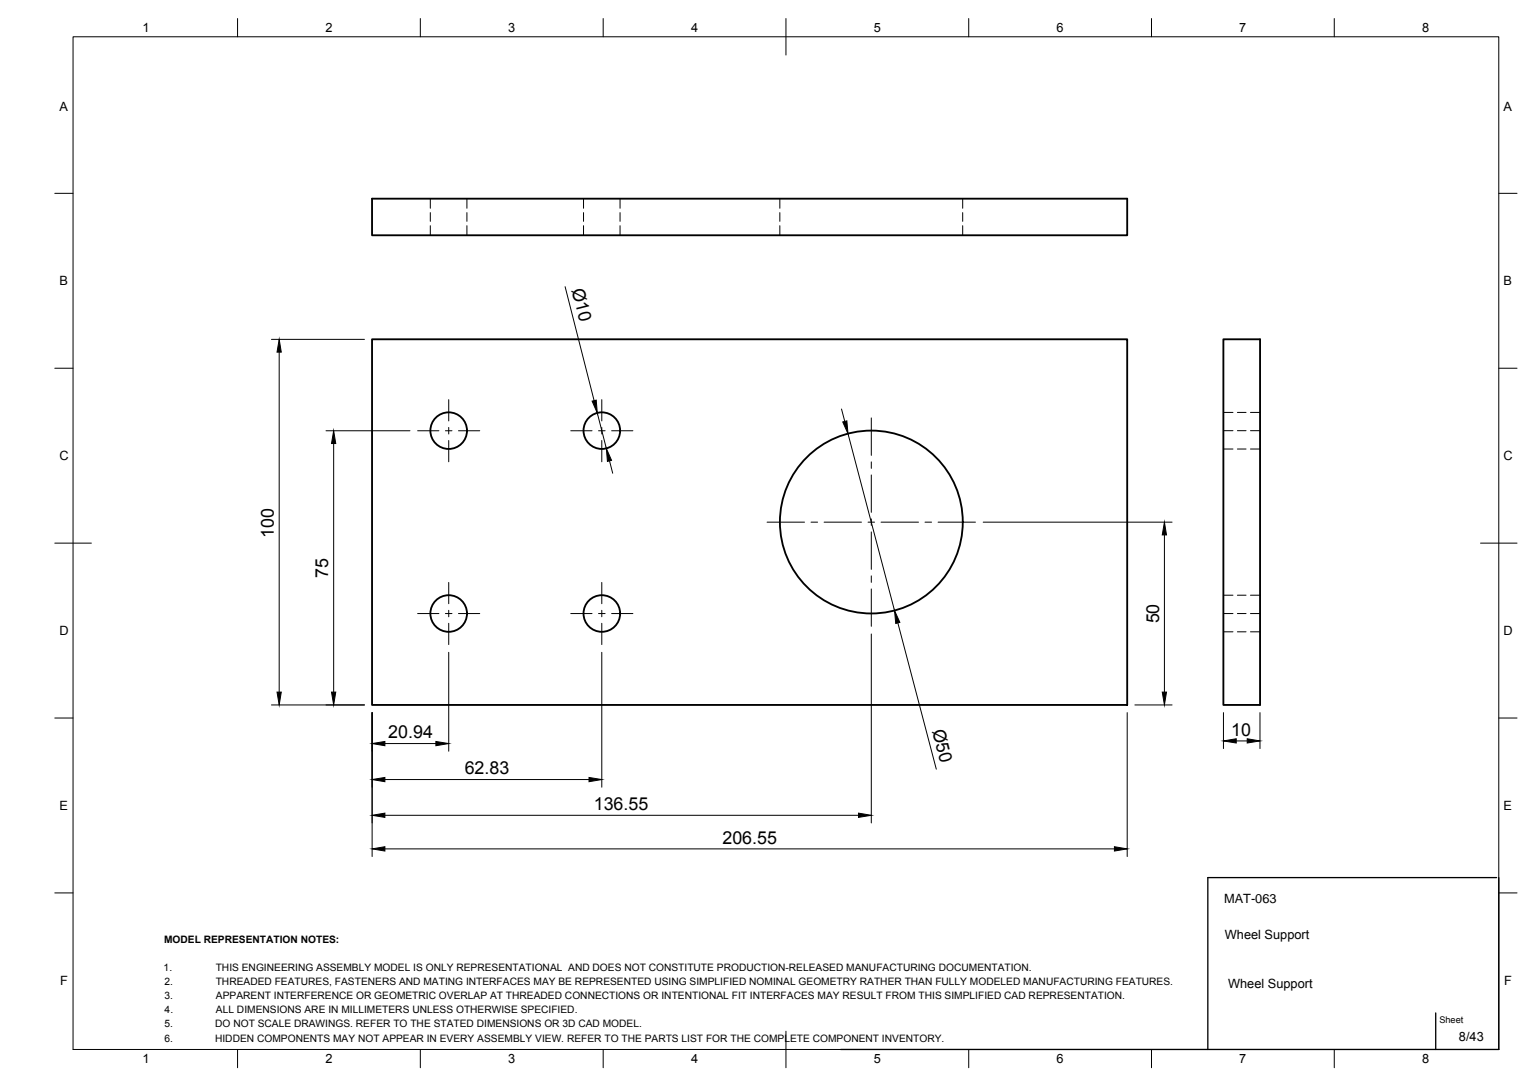
ISO-10303-21;
HEADER;
/* Generated by software containing ST-Developer
 * from STEP Tools, Inc. (www.steptools.com) 
 */

FILE_DESCRIPTION(
/* description */ (''),
/* implementation_level */ '2;1');

FILE_NAME(
/* name */ 'Wheel Support.step',
/* time_stamp */ '2026-10-24T09:43:01-07:00',
/* author */ (''),
/* organization */ (''),
/* preprocessor_version */ 'ST-DEVELOPER v20.2',
/* originating_system */ 'Autodesk Translation Framework v15.15.0.0',
/* authorisation */ '');

FILE_SCHEMA (('AUTOMOTIVE_DESIGN { 1 0 10303 214 3 1 1 }'));
ENDSEC;

DATA;
#10=MECHANICAL_DESIGN_GEOMETRIC_PRESENTATION_REPRESENTATION('',(#278),#11112);
#212=SHAPE_REPRESENTATION_RELATIONSHIP('SRR','None',#11235,#245);
#245=ADVANCED_BREP_SHAPE_REPRESENTATION('',(#311),#11080);
#278=STYLED_ITEM('',(#11426),#311);
#311=MANIFOLD_SOLID_BREP('Wheel Support',#6015);
#383=FACE_BOUND('',#1183,.T.);
#384=FACE_BOUND('',#1184,.T.);
#385=FACE_BOUND('',#1185,.T.);
#386=FACE_BOUND('',#1186,.T.);
#387=FACE_BOUND('',#1187,.T.);
#388=FACE_BOUND('',#1189,.T.);
#389=FACE_BOUND('',#1190,.T.);
#390=FACE_BOUND('',#1191,.T.);
#391=FACE_BOUND('',#1192,.T.);
#392=FACE_BOUND('',#1193,.T.);
#524=PLANE('',#6661);
#525=PLANE('',#6666);
#526=PLANE('',#6675);
#527=PLANE('',#6676);
#528=PLANE('',#6677);
#529=PLANE('',#6678);
#773=FACE_OUTER_BOUND('',#1181,.T.);
#774=FACE_OUTER_BOUND('',#1182,.T.);
#775=FACE_OUTER_BOUND('',#1188,.T.);
#776=FACE_OUTER_BOUND('',#1194,.T.);
#777=FACE_OUTER_BOUND('',#1195,.T.);
#778=FACE_OUTER_BOUND('',#1196,.T.);
#779=FACE_OUTER_BOUND('',#1197,.T.);
#780=FACE_OUTER_BOUND('',#1198,.T.);
#781=FACE_OUTER_BOUND('',#1199,.T.);
#782=FACE_OUTER_BOUND('',#1200,.T.);
#783=FACE_OUTER_BOUND('',#1201,.T.);
#1181=EDGE_LOOP('',(#4377,#4378,#4379,#4380));
#1182=EDGE_LOOP('',(#4381,#4382,#4383,#4384));
#1183=EDGE_LOOP('',(#4385));
#1184=EDGE_LOOP('',(#4386));
#1185=EDGE_LOOP('',(#4387));
#1186=EDGE_LOOP('',(#4388));
#1187=EDGE_LOOP('',(#4389));
#1188=EDGE_LOOP('',(#4390,#4391,#4392,#4393));
#1189=EDGE_LOOP('',(#4394));
#1190=EDGE_LOOP('',(#4395));
#1191=EDGE_LOOP('',(#4396));
#1192=EDGE_LOOP('',(#4397));
#1193=EDGE_LOOP('',(#4398));
#1194=EDGE_LOOP('',(#4399,#4400,#4401,#4402));
#1195=EDGE_LOOP('',(#4403,#4404,#4405,#4406));
#1196=EDGE_LOOP('',(#4407,#4408,#4409,#4410));
#1197=EDGE_LOOP('',(#4411,#4412,#4413,#4414));
#1198=EDGE_LOOP('',(#4415,#4416,#4417,#4418));
#1199=EDGE_LOOP('',(#4419,#4420,#4421,#4422));
#1200=EDGE_LOOP('',(#4423,#4424,#4425,#4426));
#1201=EDGE_LOOP('',(#4427,#4428,#4429,#4430));
#1626=LINE('',#9780,#1985);
#1627=LINE('',#9785,#1986);
#1628=LINE('',#9787,#1987);
#1629=LINE('',#9789,#1988);
#1630=LINE('',#9790,#1989);
#1631=LINE('',#9802,#1990);
#1632=LINE('',#9804,#1991);
#1633=LINE('',#9806,#1992);
#1634=LINE('',#9807,#1993);
#1635=LINE('',#9817,#1994);
#1636=LINE('',#9819,#1995);
#1637=LINE('',#9821,#1996);
#1638=LINE('',#9823,#1997);
#1639=LINE('',#9825,#1998);
#1640=LINE('',#9826,#1999);
#1641=LINE('',#9828,#2000);
#1642=LINE('',#9830,#2001);
#1985=VECTOR('',#7834,0.005);
#1986=VECTOR('',#7839,0.01);
#1987=VECTOR('',#7840,0.01);
#1988=VECTOR('',#7841,0.01);
#1989=VECTOR('',#7842,0.01);
#1990=VECTOR('',#7853,0.01);
#1991=VECTOR('',#7854,0.01);
#1992=VECTOR('',#7855,0.01);
#1993=VECTOR('',#7856,0.01);
#1994=VECTOR('',#7867,0.005);
#1995=VECTOR('',#7870,0.005);
#1996=VECTOR('',#7873,0.025);
#1997=VECTOR('',#7876,0.005);
#1998=VECTOR('',#7879,0.01);
#1999=VECTOR('',#7880,0.01);
#2000=VECTOR('',#7883,0.01);
#2001=VECTOR('',#7886,0.01);
#2420=CIRCLE('',#6659,0.005);
#2421=CIRCLE('',#6660,0.005);
#2422=CIRCLE('',#6662,0.005);
#2423=CIRCLE('',#6663,0.025);
#2424=CIRCLE('',#6664,0.005);
#2425=CIRCLE('',#6665,0.005);
#2426=CIRCLE('',#6667,0.005);
#2427=CIRCLE('',#6668,0.025);
#2428=CIRCLE('',#6669,0.005);
#2429=CIRCLE('',#6670,0.005);
#2814=VERTEX_POINT('',#9777);
#2815=VERTEX_POINT('',#9779);
#2816=VERTEX_POINT('',#9783);
#2817=VERTEX_POINT('',#9784);
#2818=VERTEX_POINT('',#9786);
#2819=VERTEX_POINT('',#9788);
#2820=VERTEX_POINT('',#9791);
#2821=VERTEX_POINT('',#9793);
#2822=VERTEX_POINT('',#9795);
#2823=VERTEX_POINT('',#9797);
#2824=VERTEX_POINT('',#9800);
#2825=VERTEX_POINT('',#9801);
#2826=VERTEX_POINT('',#9803);
#2827=VERTEX_POINT('',#9805);
#2828=VERTEX_POINT('',#9808);
#2829=VERTEX_POINT('',#9810);
#2830=VERTEX_POINT('',#9812);
#2831=VERTEX_POINT('',#9814);
#3392=EDGE_CURVE('',#2814,#2814,#2420,.T.);
#3393=EDGE_CURVE('',#2814,#2815,#1626,.T.);
#3394=EDGE_CURVE('',#2815,#2815,#2421,.F.);
#3395=EDGE_CURVE('',#2816,#2817,#1627,.T.);
#3396=EDGE_CURVE('',#2818,#2816,#1628,.T.);
#3397=EDGE_CURVE('',#2819,#2818,#1629,.T.);
#3398=EDGE_CURVE('',#2817,#2819,#1630,.T.);
#3399=EDGE_CURVE('',#2820,#2820,#2422,.T.);
#3400=EDGE_CURVE('',#2821,#2821,#2423,.T.);
#3401=EDGE_CURVE('',#2822,#2822,#2424,.T.);
#3402=EDGE_CURVE('',#2823,#2823,#2425,.T.);
#3403=EDGE_CURVE('',#2824,#2825,#1631,.T.);
#3404=EDGE_CURVE('',#2825,#2826,#1632,.T.);
#3405=EDGE_CURVE('',#2826,#2827,#1633,.T.);
#3406=EDGE_CURVE('',#2827,#2824,#1634,.T.);
#3407=EDGE_CURVE('',#2828,#2828,#2426,.T.);
#3408=EDGE_CURVE('',#2829,#2829,#2427,.T.);
#3409=EDGE_CURVE('',#2830,#2830,#2428,.T.);
#3410=EDGE_CURVE('',#2831,#2831,#2429,.T.);
#3411=EDGE_CURVE('',#2831,#2823,#1635,.T.);
#3412=EDGE_CURVE('',#2828,#2822,#1636,.T.);
#3413=EDGE_CURVE('',#2829,#2821,#1637,.T.);
#3414=EDGE_CURVE('',#2830,#2820,#1638,.T.);
#3415=EDGE_CURVE('',#2818,#2824,#1639,.T.);
#3416=EDGE_CURVE('',#2825,#2816,#1640,.T.);
#3417=EDGE_CURVE('',#2827,#2819,#1641,.T.);
#3418=EDGE_CURVE('',#2826,#2817,#1642,.T.);
#4377=ORIENTED_EDGE('',*,*,#3392,.F.);
#4378=ORIENTED_EDGE('',*,*,#3393,.T.);
#4379=ORIENTED_EDGE('',*,*,#3394,.F.);
#4380=ORIENTED_EDGE('',*,*,#3393,.F.);
#4381=ORIENTED_EDGE('',*,*,#3395,.F.);
#4382=ORIENTED_EDGE('',*,*,#3396,.F.);
#4383=ORIENTED_EDGE('',*,*,#3397,.F.);
#4384=ORIENTED_EDGE('',*,*,#3398,.F.);
#4385=ORIENTED_EDGE('',*,*,#3394,.T.);
#4386=ORIENTED_EDGE('',*,*,#3399,.F.);
#4387=ORIENTED_EDGE('',*,*,#3400,.F.);
#4388=ORIENTED_EDGE('',*,*,#3401,.F.);
#4389=ORIENTED_EDGE('',*,*,#3402,.F.);
#4390=ORIENTED_EDGE('',*,*,#3403,.T.);
#4391=ORIENTED_EDGE('',*,*,#3404,.T.);
#4392=ORIENTED_EDGE('',*,*,#3405,.T.);
#4393=ORIENTED_EDGE('',*,*,#3406,.T.);
#4394=ORIENTED_EDGE('',*,*,#3392,.T.);
#4395=ORIENTED_EDGE('',*,*,#3407,.T.);
#4396=ORIENTED_EDGE('',*,*,#3408,.T.);
#4397=ORIENTED_EDGE('',*,*,#3409,.T.);
#4398=ORIENTED_EDGE('',*,*,#3410,.T.);
#4399=ORIENTED_EDGE('',*,*,#3410,.F.);
#4400=ORIENTED_EDGE('',*,*,#3411,.T.);
#4401=ORIENTED_EDGE('',*,*,#3402,.T.);
#4402=ORIENTED_EDGE('',*,*,#3411,.F.);
#4403=ORIENTED_EDGE('',*,*,#3407,.F.);
#4404=ORIENTED_EDGE('',*,*,#3412,.T.);
#4405=ORIENTED_EDGE('',*,*,#3401,.T.);
#4406=ORIENTED_EDGE('',*,*,#3412,.F.);
#4407=ORIENTED_EDGE('',*,*,#3408,.F.);
#4408=ORIENTED_EDGE('',*,*,#3413,.T.);
#4409=ORIENTED_EDGE('',*,*,#3400,.T.);
#4410=ORIENTED_EDGE('',*,*,#3413,.F.);
#4411=ORIENTED_EDGE('',*,*,#3409,.F.);
#4412=ORIENTED_EDGE('',*,*,#3414,.T.);
#4413=ORIENTED_EDGE('',*,*,#3399,.T.);
#4414=ORIENTED_EDGE('',*,*,#3414,.F.);
#4415=ORIENTED_EDGE('',*,*,#3415,.F.);
#4416=ORIENTED_EDGE('',*,*,#3396,.T.);
#4417=ORIENTED_EDGE('',*,*,#3416,.F.);
#4418=ORIENTED_EDGE('',*,*,#3403,.F.);
#4419=ORIENTED_EDGE('',*,*,#3397,.T.);
#4420=ORIENTED_EDGE('',*,*,#3415,.T.);
#4421=ORIENTED_EDGE('',*,*,#3406,.F.);
#4422=ORIENTED_EDGE('',*,*,#3417,.T.);
#4423=ORIENTED_EDGE('',*,*,#3398,.T.);
#4424=ORIENTED_EDGE('',*,*,#3417,.F.);
#4425=ORIENTED_EDGE('',*,*,#3405,.F.);
#4426=ORIENTED_EDGE('',*,*,#3418,.T.);
#4427=ORIENTED_EDGE('',*,*,#3416,.T.);
#4428=ORIENTED_EDGE('',*,*,#3395,.T.);
#4429=ORIENTED_EDGE('',*,*,#3418,.F.);
#4430=ORIENTED_EDGE('',*,*,#3404,.F.);
#5543=CYLINDRICAL_SURFACE('',#6658,0.005);
#5544=CYLINDRICAL_SURFACE('',#6671,0.005);
#5545=CYLINDRICAL_SURFACE('',#6672,0.005);
#5546=CYLINDRICAL_SURFACE('',#6673,0.025);
#5547=CYLINDRICAL_SURFACE('',#6674,0.005);
#5746=ADVANCED_FACE('',(#773),#5543,.F.);
#5747=ADVANCED_FACE('',(#774,#383,#384,#385,#386,#387),#524,.F.);
#5748=ADVANCED_FACE('',(#775,#388,#389,#390,#391,#392),#525,.T.);
#5749=ADVANCED_FACE('',(#776),#5544,.F.);
#5750=ADVANCED_FACE('',(#777),#5545,.F.);
#5751=ADVANCED_FACE('',(#778),#5546,.F.);
#5752=ADVANCED_FACE('',(#779),#5547,.F.);
#5753=ADVANCED_FACE('',(#780),#526,.F.);
#5754=ADVANCED_FACE('',(#781),#527,.T.);
#5755=ADVANCED_FACE('',(#782),#528,.T.);
#5756=ADVANCED_FACE('',(#783),#529,.F.);
#6015=CLOSED_SHELL('',(#5746,#5747,#5748,#5749,#5750,#5751,#5752,#5753,
#5754,#5755,#5756));
#6657=AXIS2_PLACEMENT_3D('',#9775,#7828,#7829);
#6658=AXIS2_PLACEMENT_3D('',#9776,#7830,#7831);
#6659=AXIS2_PLACEMENT_3D('',#9778,#7832,#7833);
#6660=AXIS2_PLACEMENT_3D('',#9781,#7835,#7836);
#6661=AXIS2_PLACEMENT_3D('',#9782,#7837,#7838);
#6662=AXIS2_PLACEMENT_3D('',#9792,#7843,#7844);
#6663=AXIS2_PLACEMENT_3D('',#9794,#7845,#7846);
#6664=AXIS2_PLACEMENT_3D('',#9796,#7847,#7848);
#6665=AXIS2_PLACEMENT_3D('',#9798,#7849,#7850);
#6666=AXIS2_PLACEMENT_3D('',#9799,#7851,#7852);
#6667=AXIS2_PLACEMENT_3D('',#9809,#7857,#7858);
#6668=AXIS2_PLACEMENT_3D('',#9811,#7859,#7860);
#6669=AXIS2_PLACEMENT_3D('',#9813,#7861,#7862);
#6670=AXIS2_PLACEMENT_3D('',#9815,#7863,#7864);
#6671=AXIS2_PLACEMENT_3D('',#9816,#7865,#7866);
#6672=AXIS2_PLACEMENT_3D('',#9818,#7868,#7869);
#6673=AXIS2_PLACEMENT_3D('',#9820,#7871,#7872);
#6674=AXIS2_PLACEMENT_3D('',#9822,#7874,#7875);
#6675=AXIS2_PLACEMENT_3D('',#9824,#7877,#7878);
#6676=AXIS2_PLACEMENT_3D('',#9827,#7881,#7882);
#6677=AXIS2_PLACEMENT_3D('',#9829,#7884,#7885);
#6678=AXIS2_PLACEMENT_3D('',#9831,#7887,#7888);
#7828=DIRECTION('axis',(0.,0.,1.));
#7829=DIRECTION('refdir',(1.,0.,0.));
#7830=DIRECTION('center_axis',(-1.,0.,0.));
#7831=DIRECTION('ref_axis',(0.,0.,1.));
#7832=DIRECTION('center_axis',(-1.,0.,0.));
#7833=DIRECTION('ref_axis',(0.,0.,1.));
#7834=DIRECTION('',(-1.,0.,0.));
#7835=DIRECTION('center_axis',(-1.,0.,0.));
#7836=DIRECTION('ref_axis',(0.,0.,1.));
#7837=DIRECTION('center_axis',(1.,0.,0.));
#7838=DIRECTION('ref_axis',(0.,0.,-1.));
#7839=DIRECTION('',(0.,-1.,0.));
#7840=DIRECTION('',(0.,0.,1.));
#7841=DIRECTION('',(0.,1.,0.));
#7842=DIRECTION('',(0.,0.,-1.));
#7843=DIRECTION('center_axis',(-1.,0.,0.));
#7844=DIRECTION('ref_axis',(0.,0.,1.));
#7845=DIRECTION('center_axis',(-1.,0.,0.));
#7846=DIRECTION('ref_axis',(0.,0.,1.));
#7847=DIRECTION('center_axis',(-1.,0.,0.));
#7848=DIRECTION('ref_axis',(0.,0.,1.));
#7849=DIRECTION('center_axis',(-1.,0.,0.));
#7850=DIRECTION('ref_axis',(0.,0.,1.));
#7851=DIRECTION('center_axis',(1.,0.,0.));
#7852=DIRECTION('ref_axis',(0.,0.,-1.));
#7853=DIRECTION('',(0.,0.,1.));
#7854=DIRECTION('',(0.,-1.,0.));
#7855=DIRECTION('',(0.,0.,-1.));
#7856=DIRECTION('',(0.,1.,0.));
#7857=DIRECTION('center_axis',(-1.,0.,0.));
#7858=DIRECTION('ref_axis',(0.,0.,1.));
#7859=DIRECTION('center_axis',(-1.,0.,0.));
#7860=DIRECTION('ref_axis',(0.,0.,1.));
#7861=DIRECTION('center_axis',(-1.,0.,0.));
#7862=DIRECTION('ref_axis',(0.,0.,1.));
#7863=DIRECTION('center_axis',(-1.,0.,0.));
#7864=DIRECTION('ref_axis',(0.,0.,1.));
#7865=DIRECTION('center_axis',(-1.,0.,0.));
#7866=DIRECTION('ref_axis',(0.,0.,1.));
#7867=DIRECTION('',(-1.,0.,0.));
#7868=DIRECTION('center_axis',(-1.,0.,0.));
#7869=DIRECTION('ref_axis',(0.,0.,1.));
#7870=DIRECTION('',(-1.,0.,0.));
#7871=DIRECTION('center_axis',(-1.,0.,0.));
#7872=DIRECTION('ref_axis',(0.,0.,1.));
#7873=DIRECTION('',(-1.,0.,0.));
#7874=DIRECTION('center_axis',(-1.,0.,0.));
#7875=DIRECTION('ref_axis',(0.,0.,1.));
#7876=DIRECTION('',(-1.,0.,0.));
#7877=DIRECTION('center_axis',(0.,-1.,0.));
#7878=DIRECTION('ref_axis',(0.,0.,-1.));
#7879=DIRECTION('',(1.,0.,0.));
#7880=DIRECTION('',(-1.,0.,0.));
#7881=DIRECTION('center_axis',(1.43238595632038E-16,8.66263247203385E-18,
-1.));
#7882=DIRECTION('ref_axis',(-1.,7.27189582693585E-50,-1.43238595632038E-16));
#7883=DIRECTION('',(-1.,0.,0.));
#7884=DIRECTION('center_axis',(-1.18952466411614E-17,-1.,-2.57730345002263E-17));
#7885=DIRECTION('ref_axis',(-1.39638038884726E-50,2.57730345002263E-17,
-1.));
#7886=DIRECTION('',(-1.,0.,0.));
#7887=DIRECTION('center_axis',(-1.43238595632038E-16,-8.66263247203385E-18,
-1.));
#7888=DIRECTION('ref_axis',(-1.,7.27189582693585E-50,1.43238595632038E-16));
#9775=CARTESIAN_POINT('',(0.,0.,0.));
#9776=CARTESIAN_POINT('Origin',(0.51,-0.312833309,-0.025));
#9777=CARTESIAN_POINT('',(0.51,-0.312833309,-0.03));
#9778=CARTESIAN_POINT('Origin',(0.51,-0.312833309,-0.025));
#9779=CARTESIAN_POINT('',(0.5,-0.312833309,-0.03));
#9780=CARTESIAN_POINT('',(0.51,-0.312833309,-0.03));
#9781=CARTESIAN_POINT('Origin',(0.5,-0.312833309,-0.025));
#9782=CARTESIAN_POINT('Origin',(0.5,-0.353273650499999,5.93275428784068E-18));
#9783=CARTESIAN_POINT('',(0.500000000000024,-0.250000000000504,0.0499999999998374));
#9784=CARTESIAN_POINT('',(0.500000000000024,-0.456547300999497,0.0499999999998374));
#9785=CARTESIAN_POINT('',(0.5,-0.250000000038728,0.05));
#9786=CARTESIAN_POINT('',(0.500000000000024,-0.250000000000504,-0.0499999999998374));
#9787=CARTESIAN_POINT('',(0.5,-0.25,-0.0499999999875));
#9788=CARTESIAN_POINT('',(0.500000000000037,-0.456547300999497,-0.0499999999996342));
#9789=CARTESIAN_POINT('',(0.5,-0.456547300974182,-0.05));
#9790=CARTESIAN_POINT('',(0.5,-0.456547301,0.0499999999875));
#9791=CARTESIAN_POINT('',(0.5,-0.270944436,0.02));
#9792=CARTESIAN_POINT('Origin',(0.5,-0.270944436,0.025));
#9793=CARTESIAN_POINT('',(0.5,-0.386547301,-0.025));
#9794=CARTESIAN_POINT('Origin',(0.5,-0.386547301,0.));
#9795=CARTESIAN_POINT('',(0.5,-0.270944436,-0.03));
#9796=CARTESIAN_POINT('Origin',(0.5,-0.270944436,-0.025));
#9797=CARTESIAN_POINT('',(0.5,-0.312833309,0.02));
#9798=CARTESIAN_POINT('Origin',(0.5,-0.312833309,0.025));
#9799=CARTESIAN_POINT('Origin',(0.51,-0.353273650499999,5.93275428784068E-18));
#9800=CARTESIAN_POINT('',(0.509999999999963,-0.250000000000504,-0.0499999999996342));
#9801=CARTESIAN_POINT('',(0.509999999999963,-0.250000000000504,0.0499999999996342));
#9802=CARTESIAN_POINT('',(0.51,-0.25,-0.04999999998125));
#9803=CARTESIAN_POINT('',(0.509999999999976,-0.456547300999497,0.0499999999998374));
#9804=CARTESIAN_POINT('',(0.51,-0.250000000025819,0.05));
#9805=CARTESIAN_POINT('',(0.509999999999963,-0.456547300999497,-0.0499999999996342));
#9806=CARTESIAN_POINT('',(0.51,-0.456547301,0.0499999999875));
#9807=CARTESIAN_POINT('',(0.51,-0.456547300974182,-0.05));
#9808=CARTESIAN_POINT('',(0.51,-0.270944436,-0.03));
#9809=CARTESIAN_POINT('Origin',(0.51,-0.270944436,-0.025));
#9810=CARTESIAN_POINT('',(0.51,-0.386547301,-0.025));
#9811=CARTESIAN_POINT('Origin',(0.51,-0.386547301,0.));
#9812=CARTESIAN_POINT('',(0.51,-0.270944436,0.02));
#9813=CARTESIAN_POINT('Origin',(0.51,-0.270944436,0.025));
#9814=CARTESIAN_POINT('',(0.51,-0.312833309,0.02));
#9815=CARTESIAN_POINT('Origin',(0.51,-0.312833309,0.025));
#9816=CARTESIAN_POINT('Origin',(0.51,-0.312833309,0.025));
#9817=CARTESIAN_POINT('',(0.51,-0.312833309,0.02));
#9818=CARTESIAN_POINT('Origin',(0.51,-0.270944436,-0.025));
#9819=CARTESIAN_POINT('',(0.51,-0.270944436,-0.03));
#9820=CARTESIAN_POINT('Origin',(0.51,-0.386547301,0.));
#9821=CARTESIAN_POINT('',(0.51,-0.386547301,-0.025));
#9822=CARTESIAN_POINT('Origin',(0.51,-0.270944436,0.025));
#9823=CARTESIAN_POINT('',(0.51,-0.270944436,0.02));
#9824=CARTESIAN_POINT('Origin',(0.505,-0.25,5.93275428784068E-18));
#9825=CARTESIAN_POINT('',(0.500000000000001,-0.25,-0.05));
#9826=CARTESIAN_POINT('',(0.510000000000001,-0.25,0.05));
#9827=CARTESIAN_POINT('Origin',(0.505,-0.3532736505,-0.05));
#9828=CARTESIAN_POINT('',(0.510000000000001,-0.456547301,-0.05));
#9829=CARTESIAN_POINT('Origin',(0.505,-0.456547301000001,5.93275428784068E-18));
#9830=CARTESIAN_POINT('',(0.510000000000001,-0.456547301000001,0.05));
#9831=CARTESIAN_POINT('Origin',(0.505,-0.3532736505,0.05));
#11041=UNCERTAINTY_MEASURE_WITH_UNIT(LENGTH_MEASURE(1.E-5),#11113,
'DISTANCE_ACCURACY_VALUE',
'Maximum model space distance between geometric entities at asserted c
onnectivities');
#11073=UNCERTAINTY_MEASURE_WITH_UNIT(LENGTH_MEASURE(1.E-5),#11113,
'DISTANCE_ACCURACY_VALUE',
'Maximum model space distance between geometric entities at asserted c
onnectivities');
#11080=(
GEOMETRIC_REPRESENTATION_CONTEXT(3)
GLOBAL_UNCERTAINTY_ASSIGNED_CONTEXT((#11041))
GLOBAL_UNIT_ASSIGNED_CONTEXT((#11113,#11114,#11115))
REPRESENTATION_CONTEXT('','3D')
);
#11112=(
GEOMETRIC_REPRESENTATION_CONTEXT(3)
GLOBAL_UNCERTAINTY_ASSIGNED_CONTEXT((#11073))
GLOBAL_UNIT_ASSIGNED_CONTEXT((#11113,#11114,#11115))
REPRESENTATION_CONTEXT('','3D')
);
#11113=(
LENGTH_UNIT()
NAMED_UNIT(*)
SI_UNIT($,.METRE.)
);
#11114=(
NAMED_UNIT(*)
PLANE_ANGLE_UNIT()
SI_UNIT($,.RADIAN.)
);
#11115=(
NAMED_UNIT(*)
SI_UNIT($,.STERADIAN.)
SOLID_ANGLE_UNIT()
);
#11122=SHAPE_DEFINITION_REPRESENTATION(#11160,#11235);
#11160=PRODUCT_DEFINITION_SHAPE('',$,#11274);
#11235=SHAPE_REPRESENTATION('',(#6657),#11080);
#11267=PRODUCT_DEFINITION_CONTEXT('part definition',#11383,'design');
#11274=PRODUCT_DEFINITION('Wheel Support','Wheel Support',#11312,#11267);
#11312=PRODUCT_DEFINITION_FORMATION('',$,#11391);
#11383=APPLICATION_CONTEXT(
'Core Data for Automotive Mechanical Design Process');
#11384=PRODUCT_CONTEXT('part definition',#11383,'mechanical');
#11391=PRODUCT('Wheel Support','Wheel Support',
'wheel_sup__ DE    10163',(#11384));
#11426=PRESENTATION_STYLE_ASSIGNMENT((#11430));
#11430=SURFACE_STYLE_USAGE(.BOTH.,#11434);
#11434=SURFACE_SIDE_STYLE('',(#11438));
#11438=SURFACE_STYLE_FILL_AREA(#11442);
#11442=FILL_AREA_STYLE('Opaque(202,209,238)',(#11446));
#11446=FILL_AREA_STYLE_COLOUR('Opaque(202,209,238)',#11450);
#11450=COLOUR_RGB('Opaque(202,209,238)',0.792156862745098,0.819607843137255,
0.933333333333333);
ENDSEC;
END-ISO-10303-21;
